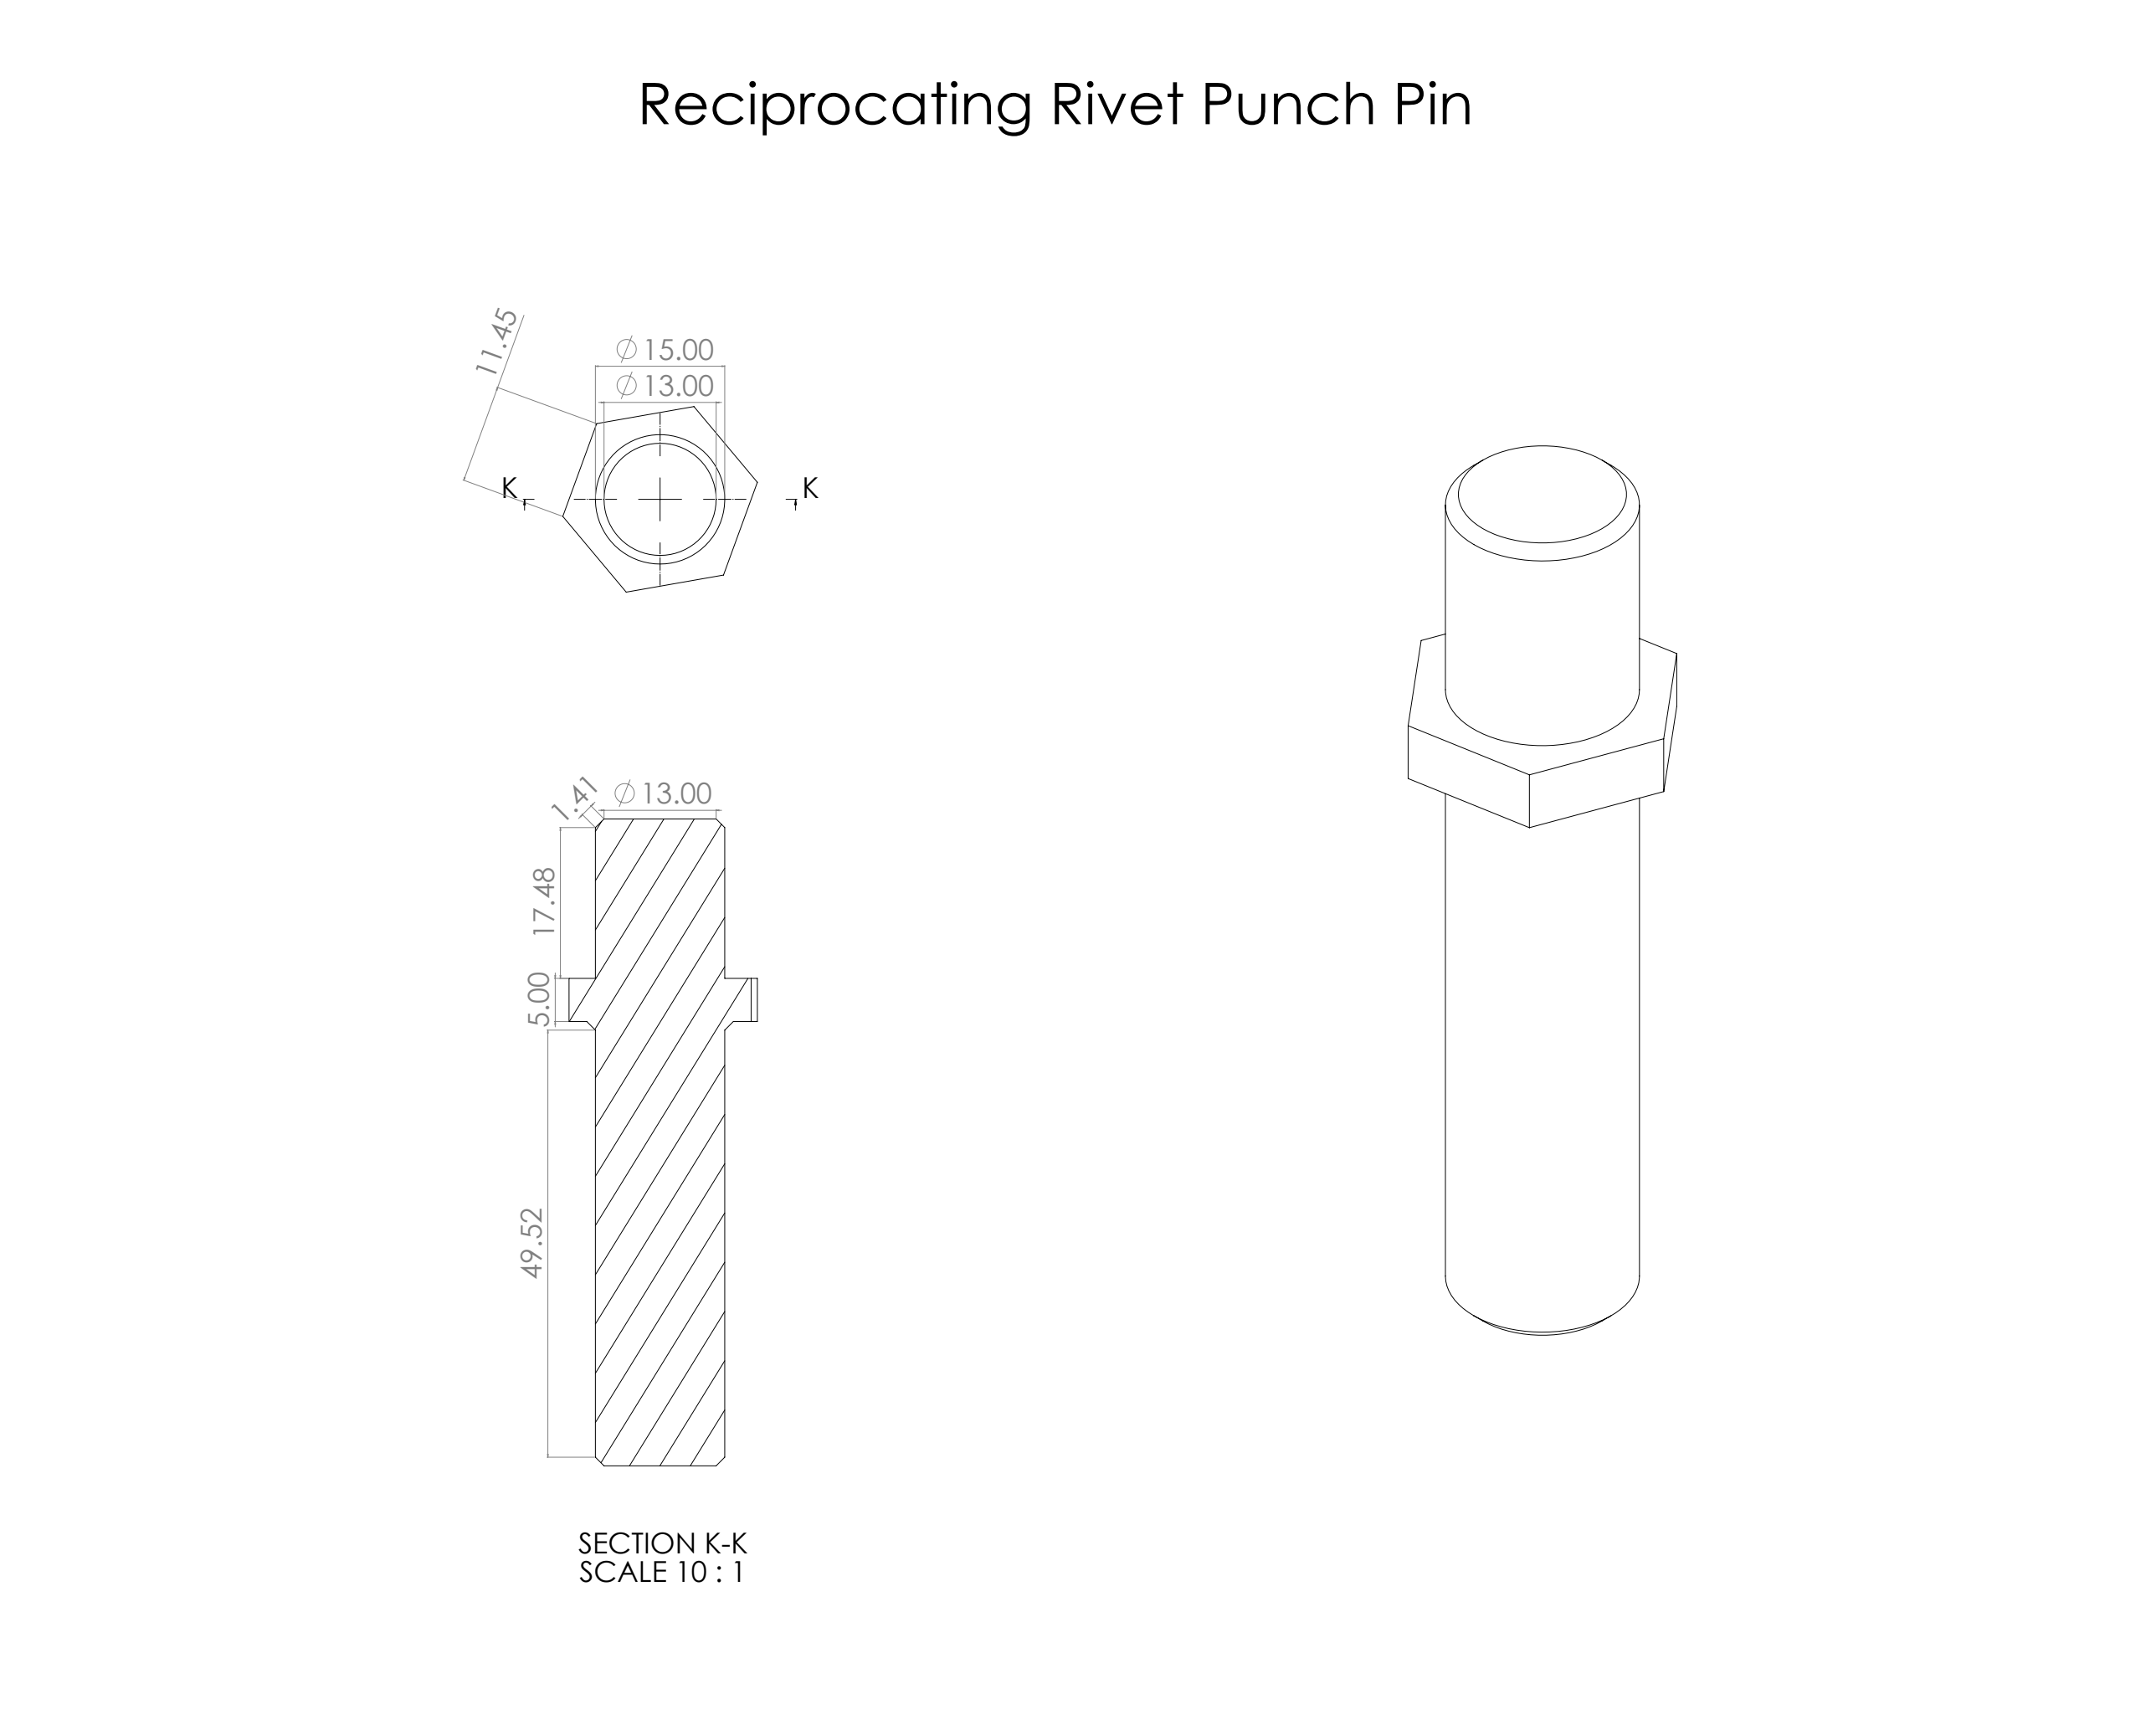
ISO-10303-21;
HEADER;
FILE_DESCRIPTION (('STEP AP214'),
    '1' );
FILE_NAME ('Reciprocating Rivet Punch Pin.step',
    '2026-10-25T20:52:49',
    ( '' ),
    ( '' ),
    'SwSTEP 2.0',
    'SolidWorks 2025',
    '' );
FILE_SCHEMA (( 'AUTOMOTIVE_DESIGN' ));
ENDSEC;

DATA;
#72=AXIS2_PLACEMENT_3D ( 'NONE', #82570, #38996, #88730 ) ;
#77=DIRECTION ( 'NONE',  ( -0.000000000000000000, 1.000000000000000000, -0.000000000000000000 ) ) ;
#121=DIRECTION ( 'NONE',  ( 0.000000000000000000, 0.7071067811865398012, 0.7071067811865552333 ) ) ;
#140=ADVANCED_BREP_SHAPE_REPRESENTATION ( '', ( #90135, #18940 ), #43137 ) ;
#206=PRODUCT_DEFINITION_CONTEXT ( 'detailed design', #57764, 'design' ) ;
#537=ORIENTED_EDGE ( 'NONE', *, *, #58978, .T. ) ;
#587=LINE ( 'NONE', #21899, #2031 ) ;
#976=EDGE_LOOP ( 'NONE', ( #39122, #15194, #45097, #86820 ) ) ;
#1223=FACE_OUTER_BOUND ( 'NONE', #24496, .T. ) ;
#1614=AXIS2_PLACEMENT_3D ( 'NONE', #18179, #47029, #23426 ) ;
#1655=EDGE_CURVE ( 'NONE', #7585, #19412, #71553, .T. ) ;
#1720=DIRECTION ( 'NONE',  ( 0.3428573139466625785, 0.000000000000000000, -0.9393874931428880526 ) ) ;
#1947=CARTESIAN_POINT ( 'NONE',  ( 208.4306832106270804, -199.2391364535880882, 0.000000000000000000 ) ) ;
#1975=DIRECTION ( 'NONE',  ( 0.000000000000000000, 0.000000000000000000, 1.000000000000000000 ) ) ;
#2031=VECTOR ( 'NONE', #28536, 1000.000000000000227 ) ;
#2392=MECHANICAL_DESIGN_GEOMETRIC_PRESENTATION_REPRESENTATION('',(#31117),#84023);
#2582=FACE_OUTER_BOUND ( 'NONE', #23796, .T. ) ;
#2617=ORIENTED_EDGE ( 'NONE', *, *, #23208, .F. ) ;
#2665=LINE ( 'NONE', #53304, #8085 ) ;
#2714=APPLICATION_CONTEXT ( 'automotive_design' ) ;
#2827=EDGE_LOOP ( 'NONE', ( #72963, #56833, #41843, #30949, #88679 ) ) ;
#3067=VERTEX_POINT ( 'NONE', #8877 ) ;
#3288=AXIS2_PLACEMENT_3D ( 'NONE', #82985, #37672, #54112 ) ;
#3409=EDGE_LOOP ( 'NONE', ( #92381, #68975, #16468, #27296, #33854 ) ) ;
#3425=AXIS2_PLACEMENT_3D ( 'NONE', #85327, #79169, #22323 ) ;
#3571=AXIS2_PLACEMENT_3D ( 'NONE', #21542, #6412, #86869 ) ;
#3656=CIRCLE ( 'NONE', #39922, 8.500000000000007105 ) ;
#3725=LINE ( 'NONE', #38757, #89716 ) ;
#3928=ORIENTED_EDGE ( 'NONE', *, *, #77906, .F. ) ;
#4091=FACE_OUTER_BOUND ( 'NONE', #61074, .T. ) ;
#4102=EDGE_CURVE ( 'NONE', #88194, #58673, #62613, .T. ) ;
#4316=AXIS2_PLACEMENT_3D ( 'NONE', #76033, #91140, #68939 ) ;
#4491=ADVANCED_FACE ( 'NONE', ( #1223 ), #8772, .T. ) ;
#4657=CIRCLE ( 'NONE', #63638, 7.500000000000012434 ) ;
#4770=EDGE_CURVE ( 'NONE', #55951, #76475, #59935, .T. ) ;
#4790=AXIS2_PLACEMENT_3D ( 'NONE', #49606, #85120, #20272 ) ;
#5162=FACE_OUTER_BOUND ( 'NONE', #92401, .T. ) ;
#5316=CLOSED_SHELL ( 'NONE', ( #16904, #77878, #27736, #81055, #54993, #32744, #82438, #11721, #85857, #23548, #86851, #61439, #15694, #44495, #51695, #4491, #81785, #83365, #7003, #77991 ) ) ;
#5328=CARTESIAN_POINT ( 'NONE',  ( 201.0776230153480526, -142.7221692137691775, -8.778910157967986905 ) ) ;
#5640=VERTEX_POINT ( 'NONE', #5328 ) ;
#5737=FACE_OUTER_BOUND ( 'NONE', #69469, .T. ) ;
#5766=VERTEX_POINT ( 'NONE', #42203 ) ;
#6030=EDGE_CURVE ( 'NONE', #93585, #33595, #3656, .T. ) ;
#6260=VERTEX_POINT ( 'NONE', #88559 ) ;
#6299=CIRCLE ( 'NONE', #4790, 7.500000000000012434 ) ;
#6412=DIRECTION ( 'NONE',  ( 0.000000000000000000, -1.000000000000000000, 0.000000000000000000 ) ) ;
#6560=CIRCLE ( 'NONE', #14137, 6.499999999999977796 ) ;
#6590=CIRCLE ( 'NONE', #11085, 7.500000000000012434 ) ;
#6657=CARTESIAN_POINT ( 'NONE',  ( 208.4306832106270804, -125.2391364535880882, -7.500000000000012434 ) ) ;
#6698=FACE_OUTER_BOUND ( 'NONE', #91473, .T. ) ;
#6794=DIRECTION ( 'NONE',  ( 8.659560562354937789E-17, -0.7071067811865472397, 0.7071067811865479058 ) ) ;
#7001=DIRECTION ( 'NONE',  ( 0.3428573139466625785, 0.000000000000000000, -0.9393874931428881636 ) ) ;
#7003=ADVANCED_FACE ( 'NONE', ( #25107 ), #30972, .T. ) ;
#7032=CARTESIAN_POINT ( 'NONE',  ( 208.4306832106270804, -124.2391364535881024, 6.500000000000033751 ) ) ;
#7127=DIRECTION ( 'NONE',  ( 0.000000000000000000, -1.000000000000000000, 0.000000000000000000 ) ) ;
#7130=DIRECTION ( 'NONE',  ( 0.000000000000000000, 0.7071067811865453523, 0.7071067811865496822 ) ) ;
#7541=EDGE_CURVE ( 'NONE', #54596, #88194, #59177, .T. ) ;
#7585=VERTEX_POINT ( 'NONE', #72013 ) ;
#7677=DIRECTION ( 'NONE',  ( 0.000000000000000000, -1.000000000000000000, 0.000000000000000000 ) ) ;
#7824=AXIS2_PLACEMENT_3D ( 'NONE', #80114, #7677, #30388 ) ;
#7846=CARTESIAN_POINT ( 'NONE',  ( 208.4306832106270804, -124.2391364535881024, 0.000000000000000000 ) ) ;
#8060=AXIS2_PLACEMENT_3D ( 'NONE', #85266, #71074, #64474 ) ;
#8085=VECTOR ( 'NONE', #1720, 1000.000000000000227 ) ;
#8088=SHAPE_REPRESENTATION_RELATIONSHIP ( 'NONE' , 'NONE' ,  #54338, #140 ) ;
#8356=DIRECTION ( 'NONE',  ( -0.9393874931428880526, 0.000000000000000000, -0.3428573139466629116 ) ) ;
#8384=PRODUCT_DEFINITION_FORMATION_WITH_SPECIFIED_SOURCE ( 'ANY', '', #15547, .NOT_KNOWN. ) ;
#8414=ORIENTED_EDGE ( 'NONE', *, *, #71951, .F. ) ;
#8515=LINE ( 'NONE', #80958, #86658 ) ;
#8772=PLANE ( 'NONE',  #50500 ) ;
#8877=CARTESIAN_POINT ( 'NONE',  ( 212.3569123273291268, -142.7221692137691775, -10.75739200365177695 ) ) ;
#9033=CYLINDRICAL_SURFACE ( 'NONE', #53545, 7.500000000000007105 ) ;
#9259=CARTESIAN_POINT ( 'NONE',  ( 208.4306832106270804, -124.2391364535881024, 0.000000000000000000 ) ) ;
#9285=EDGE_CURVE ( 'NONE', #6260, #33595, #40858, .T. ) ;
#9394=CARTESIAN_POINT ( 'NONE',  ( 204.5044540939250055, -147.7221692137691775, 10.75739200365177695 ) ) ;
#9436=DIRECTION ( 'NONE',  ( -1.000000000000000000, 0.000000000000000000, 0.000000000000000000 ) ) ;
#9489=CARTESIAN_POINT ( 'NONE',  ( 208.4306832106270804, -125.2391364535880882, 7.500000000000012434 ) ) ;
#9499=DIRECTION ( 'NONE',  ( -1.000000000000000000, 0.000000000000000000, 0.000000000000000000 ) ) ;
#9642=CIRCLE ( 'NONE', #62592, 6.500000000000033751 ) ;
#9668=CARTESIAN_POINT ( 'NONE',  ( 208.4306832106270804, -125.2391364535880882, 0.000000000000000000 ) ) ;
#9948=ORIENTED_EDGE ( 'NONE', *, *, #41512, .F. ) ;
#10028=DIRECTION ( 'NONE',  ( 0.1727706028203384314, 0.000000000000000000, 0.9849620900324524975 ) ) ;
#10210=DIRECTION ( 'NONE',  ( 1.124465274301078034E-16, 1.000000000000000000, 0.000000000000000000 ) ) ;
#10398=ORIENTED_EDGE ( 'NONE', *, *, #37113, .T. ) ;
#10664=EDGE_CURVE ( 'NONE', #76475, #64288, #20217, .T. ) ;
#10780=EDGE_CURVE ( 'NONE', #45114, #88143, #68943, .T. ) ;
#11003=ORIENTED_EDGE ( 'NONE', *, *, #10664, .F. ) ;
#11083=CYLINDRICAL_SURFACE ( 'NONE', #25795, 7.500000000000007105 ) ;
#11085=AXIS2_PLACEMENT_3D ( 'NONE', #46770, #69049, #68580 ) ;
#11101=VERTEX_POINT ( 'NONE', #43324 ) ;
#11263=EDGE_LOOP ( 'NONE', ( #75878, #62352 ) ) ;
#11601=UNCERTAINTY_MEASURE_WITH_UNIT (LENGTH_MEASURE( 1.000000000000000082E-05 ), #72501, 'distance_accuracy_value', 'NONE');
#11721=ADVANCED_FACE ( 'NONE', ( #12583, #14467 ), #20624, .T. ) ;
#11722=VERTEX_POINT ( 'NONE', #77439 ) ;
#12355=VERTEX_POINT ( 'NONE', #38848 ) ;
#12583=FACE_BOUND ( 'NONE', #70208, .T. ) ;
#12655=AXIS2_PLACEMENT_3D ( 'NONE', #19670, #75110, #76037 ) ;
#12972=EDGE_CURVE ( 'NONE', #34180, #5640, #63025, .T. ) ;
#13047=CARTESIAN_POINT ( 'NONE',  ( 215.9306832106270804, -199.2391364535880882, 9.184850993605165694E-16 ) ) ;
#13168=DIRECTION ( 'NONE',  ( -0.000000000000000000, 1.000000000000000000, -0.000000000000000000 ) ) ;
#13276=CARTESIAN_POINT ( 'NONE',  ( 208.4306832106270804, -147.7221692137691775, -8.500000000000007105 ) ) ;
#13304=LINE ( 'NONE', #27023, #54729 ) ;
#13606=CARTESIAN_POINT ( 'NONE',  ( 219.7099725226080977, -147.7221692137691775, -1.978481845683818907 ) ) ;
#13817=ORIENTED_EDGE ( 'NONE', *, *, #63823, .T. ) ;
#14137=AXIS2_PLACEMENT_3D ( 'NONE', #65588, #30978, #58466 ) ;
#14171=ORIENTED_EDGE ( 'NONE', *, *, #20803, .F. ) ;
#14349=DIRECTION ( 'NONE',  ( 0.000000000000000000, -1.000000000000000000, 0.000000000000000000 ) ) ;
#14467=FACE_OUTER_BOUND ( 'NONE', #66572, .T. ) ;
#14750=( NAMED_UNIT ( * ) SI_UNIT ( $, .STERADIAN. ) SOLID_ANGLE_UNIT ( ) );
#14841=CARTESIAN_POINT ( 'NONE',  ( 208.4306832106270804, -199.2391364535880882, -6.499999999999977796 ) ) ;
#14968=DIRECTION ( 'NONE',  ( -1.000000000000000000, 1.124465274301078034E-16, 0.000000000000000000 ) ) ;
#14996=ORIENTED_EDGE ( 'NONE', *, *, #71951, .T. ) ;
#15194=ORIENTED_EDGE ( 'NONE', *, *, #83604, .F. ) ;
#15469=CARTESIAN_POINT ( 'NONE',  ( 215.9306832106270804, -142.7221692137691775, 9.184850993605173582E-16 ) ) ;
#15547=PRODUCT ( 'Reciprocating Rivet Punch Pin', 'Reciprocating Rivet Punch Pin', '', ( #47307 ) ) ;
#15642=DIRECTION ( 'NONE',  ( -0.1727706028203382094, 0.000000000000000000, -0.9849620900324524975 ) ) ;
#15689=CARTESIAN_POINT ( 'NONE',  ( 200.9306832106270804, -198.2391364535880598, 0.000000000000000000 ) ) ;
#15694=ADVANCED_FACE ( 'NONE', ( #71880 ), #86979, .F. ) ;
#15702=VECTOR ( 'NONE', #13168, 1000.000000000000000 ) ;
#15862=EDGE_CURVE ( 'NONE', #33370, #72504, #6299, .T. ) ;
#16115=FACE_OUTER_BOUND ( 'NONE', #976, .T. ) ;
#16127=ORIENTED_EDGE ( 'NONE', *, *, #65170, .F. ) ;
#16202=CARTESIAN_POINT ( 'NONE',  ( 201.0776230153480526, -142.7221692137691775, -8.778910157967986905 ) ) ;
#16468=ORIENTED_EDGE ( 'NONE', *, *, #58978, .F. ) ;
#16556=DIRECTION ( 'NONE',  ( -0.9849620900324524975, 0.000000000000000000, 0.1727706028203382094 ) ) ;
#16904=ADVANCED_FACE ( 'NONE', ( #25374 ), #51681, .T. ) ;
#17060=ORIENTED_EDGE ( 'NONE', *, *, #41512, .T. ) ;
#17146=PLANE ( 'NONE',  #66255 ) ;
#17317=VECTOR ( 'NONE', #86922, 1000.000000000000227 ) ;
#17425=ORIENTED_EDGE ( 'NONE', *, *, #25604, .F. ) ;
#17781=CARTESIAN_POINT ( 'NONE',  ( 219.7099725226080977, -142.7221692137691775, -1.978481845683818907 ) ) ;
#17814=DIRECTION ( 'NONE',  ( 0.000000000000000000, 0.000000000000000000, -1.000000000000000000 ) ) ;
#17858=ORIENTED_EDGE ( 'NONE', *, *, #31125, .F. ) ;
#18014=DIRECTION ( 'NONE',  ( -0.6421047760857900855, 0.000000000000000000, -0.7666168903225504261 ) ) ;
#18179=CARTESIAN_POINT ( 'NONE',  ( 208.4306832106270804, -124.2391364535881024, 0.000000000000000000 ) ) ;
#18207=EDGE_CURVE ( 'NONE', #5766, #41385, #13304, .T. ) ;
#18488=DIRECTION ( 'NONE',  ( -0.000000000000000000, 1.000000000000000000, -0.000000000000000000 ) ) ;
#18617=CARTESIAN_POINT ( 'NONE',  ( 201.0776230153480526, -147.7221692137691775, -8.778910157967986905 ) ) ;
#18940=AXIS2_PLACEMENT_3D ( 'NONE', #90959, #40773, #33703 ) ;
#18953=ORIENTED_EDGE ( 'NONE', *, *, #91976, .T. ) ;
#19412=VERTEX_POINT ( 'NONE', #48154 ) ;
#19670=CARTESIAN_POINT ( 'NONE',  ( 208.4306832106270804, -198.2391364535880598, 0.000000000000000000 ) ) ;
#19762=ORIENTED_EDGE ( 'NONE', *, *, #42341, .T. ) ;
#20204=CARTESIAN_POINT ( 'NONE',  ( 208.4306832106270804, -198.2391364535880598, 0.000000000000000000 ) ) ;
#20217=CIRCLE ( 'NONE', #12655, 7.500000000000012434 ) ;
#20224=ORIENTED_EDGE ( 'NONE', *, *, #62141, .F. ) ;
#20272=DIRECTION ( 'NONE',  ( 0.000000000000000000, 0.000000000000000000, -1.000000000000000000 ) ) ;
#20412=VERTEX_POINT ( 'NONE', #23006 ) ;
#20624=PLANE ( 'NONE',  #3571 ) ;
#20706=ORIENTED_EDGE ( 'NONE', *, *, #63388, .F. ) ;
#20803=EDGE_CURVE ( 'NONE', #11722, #85835, #45229, .T. ) ;
#21161=DIRECTION ( 'NONE',  ( -0.3428573139466628561, 0.000000000000000000, 0.9393874931428880526 ) ) ;
#21282=ORIENTED_EDGE ( 'NONE', *, *, #58839, .F. ) ;
#21542=CARTESIAN_POINT ( 'NONE',  ( 0.000000000000000000, -147.7221692137691775, 0.000000000000000000 ) ) ;
#21704=VECTOR ( 'NONE', #54708, 1000.000000000000114 ) ;
#21849=( NAMED_UNIT ( * ) PLANE_ANGLE_UNIT ( ) SI_UNIT ( $, .RADIAN. ) );
#21899=CARTESIAN_POINT ( 'NONE',  ( 197.1513938986460062, -142.7221692137691775, 1.978481845683761620 ) ) ;
#22323=DIRECTION ( 'NONE',  ( 0.000000000000000000, 0.000000000000000000, -1.000000000000000000 ) ) ;
#22485=ORIENTED_EDGE ( 'NONE', *, *, #4102, .T. ) ;
#22559=DIRECTION ( 'NONE',  ( -0.3428573139466628561, 0.000000000000000000, 0.9393874931428879416 ) ) ;
#22606=LINE ( 'NONE', #73293, #53482 ) ;
#22911=EDGE_CURVE ( 'NONE', #58673, #7585, #52708, .T. ) ;
#23006=CARTESIAN_POINT ( 'NONE',  ( 215.9306832106270804, -125.2391364535880882, 9.184850993605173582E-16 ) ) ;
#23208=EDGE_CURVE ( 'NONE', #6260, #7585, #59410, .T. ) ;
#23426=DIRECTION ( 'NONE',  ( 0.000000000000000000, 0.000000000000000000, -1.000000000000000000 ) ) ;
#23548=ADVANCED_FACE ( 'NONE', ( #87872 ), #30599, .F. ) ;
#23558=EDGE_CURVE ( 'NONE', #3067, #11722, #66143, .T. ) ;
#23666=CARTESIAN_POINT ( 'NONE',  ( 208.4306832106270804, -199.2391364535880882, 0.000000000000000000 ) ) ;
#23796=EDGE_LOOP ( 'NONE', ( #2617, #58758, #77226, #53153, #79683 ) ) ;
#23934=EDGE_LOOP ( 'NONE', ( #17060, #22485, #26611, #77860, #537, #76910 ) ) ;
#24496=EDGE_LOOP ( 'NONE', ( #46361, #93472 ) ) ;
#24799=VECTOR ( 'NONE', #18488, 1000.000000000000000 ) ;
#24999=EDGE_CURVE ( 'NONE', #55951, #54596, #6560, .T. ) ;
#25002=CARTESIAN_POINT ( 'NONE',  ( 212.3569123273291268, -147.7221692137691775, -10.75739200365177695 ) ) ;
#25076=CARTESIAN_POINT ( 'NONE',  ( 215.7837434059060229, -147.7221692137691775, 8.778910157967997563 ) ) ;
#25083=CARTESIAN_POINT ( 'NONE',  ( 208.4306832106270804, -198.2391364535880598, 7.500000000000012434 ) ) ;
#25107=FACE_OUTER_BOUND ( 'NONE', #3409, .T. ) ;
#25374=FACE_OUTER_BOUND ( 'NONE', #46111, .T. ) ;
#25441=EDGE_LOOP ( 'NONE', ( #83264, #71223, #50033, #74140, #54424 ) ) ;
#25604=EDGE_CURVE ( 'NONE', #34180, #77042, #60786, .T. ) ;
#25730=CIRCLE ( 'NONE', #78678, 7.500000000000012434 ) ;
#25752=DIRECTION ( 'NONE',  ( -1.000000000000000000, 0.000000000000000000, 0.000000000000000000 ) ) ;
#25795=AXIS2_PLACEMENT_3D ( 'NONE', #61759, #90592, #25752 ) ;
#25846=DIRECTION ( 'NONE',  ( -0.6421047760857900855, 0.000000000000000000, -0.7666168903225505371 ) ) ;
#26204=VECTOR ( 'NONE', #91014, 1000.000000000000114 ) ;
#26611=ORIENTED_EDGE ( 'NONE', *, *, #22911, .T. ) ;
#26632=DIRECTION ( 'NONE',  ( 0.6421047760857910847, 0.000000000000000000, 0.7666168903225496489 ) ) ;
#26752=EDGE_CURVE ( 'NONE', #11101, #37419, #3725, .T. ) ;
#27023=CARTESIAN_POINT ( 'NONE',  ( 215.7837434059060229, -147.7221692137691775, 8.778910157967997563 ) ) ;
#27035=DIRECTION ( 'NONE',  ( 0.6421047760857910847, 0.000000000000000000, 0.7666168903225496489 ) ) ;
#27296=ORIENTED_EDGE ( 'NONE', *, *, #49214, .T. ) ;
#27646=VECTOR ( 'NONE', #73698, 1000.000000000000000 ) ;
#27736=ADVANCED_FACE ( 'NONE', ( #69867 ), #56315, .T. ) ;
#27854=DIRECTION ( 'NONE',  ( 0.9393874931428881636, 0.000000000000000000, 0.3428573139466625785 ) ) ;
#27980=DIRECTION ( 'NONE',  ( 0.000000000000000000, 0.000000000000000000, 1.000000000000000000 ) ) ;
#28464=PLANE ( 'NONE',  #35453 ) ;
#28536=DIRECTION ( 'NONE',  ( 0.3428573139466625785, 0.000000000000000000, -0.9393874931428880526 ) ) ;
#29004=CARTESIAN_POINT ( 'NONE',  ( 208.4306832106270804, -147.7221692137691775, 8.500000000000007105 ) ) ;
#30297=EDGE_CURVE ( 'NONE', #12355, #5766, #71369, .T. ) ;
#30388=DIRECTION ( 'NONE',  ( 0.000000000000000000, 0.000000000000000000, -1.000000000000000000 ) ) ;
#30404=LINE ( 'NONE', #16202, #63432 ) ;
#30467=ORIENTED_EDGE ( 'NONE', *, *, #4102, .F. ) ;
#30576=ORIENTED_EDGE ( 'NONE', *, *, #79173, .T. ) ;
#30590=DIRECTION ( 'NONE',  ( -1.000000000000000000, 0.000000000000000000, 0.000000000000000000 ) ) ;
#30599=PLANE ( 'NONE',  #41176 ) ;
#30783=AXIS2_PLACEMENT_3D ( 'NONE', #32164, #40168, #62940 ) ;
#30949=ORIENTED_EDGE ( 'NONE', *, *, #58839, .T. ) ;
#30972=CONICAL_SURFACE ( 'NONE', #65807, 8.500000000000007105, 0.7853981633974591592 ) ;
#30978=DIRECTION ( 'NONE',  ( -1.124465274301078034E-16, -1.000000000000000000, -0.000000000000000000 ) ) ;
#31117=STYLED_ITEM('',(#93752),#90135);
#31125=EDGE_CURVE ( 'NONE', #11101, #83213, #32020, .T. ) ;
#31483=CARTESIAN_POINT ( 'NONE',  ( 208.4306832106270804, -199.2391364535880882, 6.499999999999977796 ) ) ;
#31563=CIRCLE ( 'NONE', #4316, 7.500000000000012434 ) ;
#31615=ORIENTED_EDGE ( 'NONE', *, *, #12972, .T. ) ;
#31631=CARTESIAN_POINT ( 'NONE',  ( 201.0776230153480526, -147.7221692137691775, -8.778910157967986905 ) ) ;
#32020=CIRCLE ( 'NONE', #3288, 6.500000000000033751 ) ;
#32058=ORIENTED_EDGE ( 'NONE', *, *, #50406, .F. ) ;
#32164=CARTESIAN_POINT ( 'NONE',  ( 208.4306832106270804, -199.2391364535880882, 0.000000000000000000 ) ) ;
#32602=CARTESIAN_POINT ( 'NONE',  ( 197.1513938986460062, -147.7221692137691775, 1.978481845683761620 ) ) ;
#32744=ADVANCED_FACE ( 'NONE', ( #73916 ), #9033, .T. ) ;
#32799=LINE ( 'NONE', #90984, #60892 ) ;
#32962=PLANE ( 'NONE',  #72925 ) ;
#32977=ORIENTED_EDGE ( 'NONE', *, *, #20803, .T. ) ;
#33171=CARTESIAN_POINT ( 'NONE',  ( 208.4306832106270804, -147.7221692137691775, 0.000000000000000000 ) ) ;
#33370=VERTEX_POINT ( 'NONE', #48284 ) ;
#33595=VERTEX_POINT ( 'NONE', #13276 ) ;
#33703=DIRECTION ( 'NONE',  ( 1.000000000000000000, 0.000000000000000000, 0.000000000000000000 ) ) ;
#33854=ORIENTED_EDGE ( 'NONE', *, *, #37113, .F. ) ;
#34037=PLANE ( 'NONE',  #30783 ) ;
#34180=VERTEX_POINT ( 'NONE', #31631 ) ;
#34838=CARTESIAN_POINT ( 'NONE',  ( 208.4306832106270804, -199.2391364535880882, 0.000000000000000000 ) ) ;
#35128=EDGE_LOOP ( 'NONE', ( #52939, #84957, #51732, #30467, #80366 ) ) ;
#35370=AXIS2_PLACEMENT_3D ( 'NONE', #20204, #49083, #77981 ) ;
#35382=AXIS2_PLACEMENT_3D ( 'NONE', #58618, #79915, #67115 ) ;
#35453=AXIS2_PLACEMENT_3D ( 'NONE', #50704, #79592, #36028 ) ;
#35595=ORIENTED_EDGE ( 'NONE', *, *, #4770, .F. ) ;
#35872=EDGE_CURVE ( 'NONE', #88143, #5640, #587, .T. ) ;
#36028=DIRECTION ( 'NONE',  ( 0.000000000000000000, -0.000000000000000000, -1.000000000000000000 ) ) ;
#36222=CIRCLE ( 'NONE', #70980, 7.500000000000012434 ) ;
#36420=ORIENTED_EDGE ( 'NONE', *, *, #24999, .T. ) ;
#36556=CIRCLE ( 'NONE', #84942, 7.500000000000012434 ) ;
#36765=DIRECTION ( 'NONE',  ( 1.124465274301078034E-16, 1.000000000000000000, 0.000000000000000000 ) ) ;
#37113=EDGE_CURVE ( 'NONE', #33595, #93585, #74616, .T. ) ;
#37419=VERTEX_POINT ( 'NONE', #6657 ) ;
#37672=DIRECTION ( 'NONE',  ( 1.124465274301078034E-16, 1.000000000000000000, 0.000000000000000000 ) ) ;
#37692=LINE ( 'NONE', #75100, #45859 ) ;
#38198=ORIENTED_EDGE ( 'NONE', *, *, #25604, .T. ) ;
#38757=CARTESIAN_POINT ( 'NONE',  ( 208.4306832106270804, -124.2391364535881024, -6.500000000000024869 ) ) ;
#38848=CARTESIAN_POINT ( 'NONE',  ( 219.7099725226080977, -147.7221692137691775, -1.978481845683818907 ) ) ;
#38869=CARTESIAN_POINT ( 'NONE',  ( 208.4306832106270804, -125.2391364535880882, 0.000000000000000000 ) ) ;
#38898=DIRECTION ( 'NONE',  ( 0.9849620900324523864, 0.000000000000000000, -0.1727706028203384037 ) ) ;
#38996=DIRECTION ( 'NONE',  ( -0.000000000000000000, 1.000000000000000000, -0.000000000000000000 ) ) ;
#39059=DIRECTION ( 'NONE',  ( -0.3428573139466628561, 0.000000000000000000, 0.9393874931428880526 ) ) ;
#39122=ORIENTED_EDGE ( 'NONE', *, *, #81466, .T. ) ;
#39171=DIRECTION ( 'NONE',  ( -0.000000000000000000, 1.000000000000000000, -0.000000000000000000 ) ) ;
#39359=CONICAL_SURFACE ( 'NONE', #72, 8.500000000000007105, 0.7853981633974591592 ) ;
#39455=FACE_OUTER_BOUND ( 'NONE', #75250, .T. ) ;
#39550=CARTESIAN_POINT ( 'NONE',  ( 208.4306832106270804, -124.2391364535881024, 0.000000000000000000 ) ) ;
#39922=AXIS2_PLACEMENT_3D ( 'NONE', #64974, #77, #88080 ) ;
#40000=AXIS2_PLACEMENT_3D ( 'NONE', #25076, #15642, #59204 ) ;
#40032=DIRECTION ( 'NONE',  ( 0.000000000000000000, -1.000000000000000000, 0.000000000000000000 ) ) ;
#40168=DIRECTION ( 'NONE',  ( 1.124465274301078034E-16, 1.000000000000000000, 0.000000000000000000 ) ) ;
#40188=DIRECTION ( 'NONE',  ( 0.000000000000000000, 0.000000000000000000, -1.000000000000000000 ) ) ;
#40526=UNCERTAINTY_MEASURE_WITH_UNIT (LENGTH_MEASURE( 1.000000000000000082E-05 ), #42925, 'distance_accuracy_value', 'NONE');
#40649=CARTESIAN_POINT ( 'NONE',  ( 197.1513938986460062, -142.7221692137691775, 1.978481845683761620 ) ) ;
#40773=DIRECTION ( 'NONE',  ( 0.000000000000000000, 0.000000000000000000, 1.000000000000000000 ) ) ;
#40858=LINE ( 'NONE', #75475, #59487 ) ;
#41175=DIRECTION ( 'NONE',  ( 0.000000000000000000, 0.000000000000000000, -1.000000000000000000 ) ) ;
#41176=AXIS2_PLACEMENT_3D ( 'NONE', #73245, #8356, #22559 ) ;
#41289=DIRECTION ( 'NONE',  ( 0.000000000000000000, 0.000000000000000000, -1.000000000000000000 ) ) ;
#41385=VERTEX_POINT ( 'NONE', #9394 ) ;
#41512=EDGE_CURVE ( 'NONE', #64288, #88194, #6590, .T. ) ;
#41552=VECTOR ( 'NONE', #7130, 1000.000000000000227 ) ;
#41624=EDGE_CURVE ( 'NONE', #72504, #33370, #86650, .T. ) ;
#41843=ORIENTED_EDGE ( 'NONE', *, *, #77906, .T. ) ;
#42203=CARTESIAN_POINT ( 'NONE',  ( 215.7837434059060229, -147.7221692137691775, 8.778910157967997563 ) ) ;
#42341=EDGE_CURVE ( 'NONE', #12355, #11722, #78028, .T. ) ;
#42925=( LENGTH_UNIT ( ) NAMED_UNIT ( * ) SI_UNIT ( .MILLI., .METRE. ) );
#43137=( GEOMETRIC_REPRESENTATION_CONTEXT ( 3 ) GLOBAL_UNCERTAINTY_ASSIGNED_CONTEXT ( ( #11601 ) ) GLOBAL_UNIT_ASSIGNED_CONTEXT ( ( #72501, #21849, #14750 ) ) REPRESENTATION_CONTEXT ( 'NONE', 'WORKASPACE' ) );
#43211=LINE ( 'NONE', #29004, #58810 ) ;
#43324=CARTESIAN_POINT ( 'NONE',  ( 208.4306832106270804, -124.2391364535881024, -6.500000000000033751 ) ) ;
#43487=DIRECTION ( 'NONE',  ( -0.000000000000000000, 1.000000000000000000, -0.000000000000000000 ) ) ;
#43625=EDGE_LOOP ( 'NONE', ( #50959, #20224, #17425, #31615 ) ) ;
#44040=FACE_BOUND ( 'NONE', #11263, .T. ) ;
#44114=AXIS2_PLACEMENT_3D ( 'NONE', #92685, #27854, #7001 ) ;
#44495=ADVANCED_FACE ( 'NONE', ( #73969 ), #17146, .F. ) ;
#44749=VECTOR ( 'NONE', #43487, 1000.000000000000000 ) ;
#44966=PLANE ( 'NONE',  #40000 ) ;
#45097=ORIENTED_EDGE ( 'NONE', *, *, #18207, .F. ) ;
#45114=VERTEX_POINT ( 'NONE', #68746 ) ;
#45229=LINE ( 'NONE', #17781, #77447 ) ;
#45323=EDGE_CURVE ( 'NONE', #33370, #62133, #87134, .T. ) ;
#45592=DIRECTION ( 'NONE',  ( 1.124465274301078034E-16, 1.000000000000000000, 0.000000000000000000 ) ) ;
#45787=VECTOR ( 'NONE', #45592, 1000.000000000000000 ) ;
#45859=VECTOR ( 'NONE', #10210, 1000.000000000000000 ) ;
#45922=SHAPE_DEFINITION_REPRESENTATION ( #58649, #54338 ) ;
#46013=CARTESIAN_POINT ( 'NONE',  ( 201.0776230153480526, -147.7221692137691775, -8.778910157967986905 ) ) ;
#46111=EDGE_LOOP ( 'NONE', ( #90811, #30576, #3928, #90125, #72298 ) ) ;
#46238=ORIENTED_EDGE ( 'NONE', *, *, #10780, .F. ) ;
#46295=ORIENTED_EDGE ( 'NONE', *, *, #49739, .F. ) ;
#46361=ORIENTED_EDGE ( 'NONE', *, *, #31125, .T. ) ;
#46453=ORIENTED_EDGE ( 'NONE', *, *, #7541, .T. ) ;
#46714=EDGE_CURVE ( 'NONE', #58673, #76475, #31563, .T. ) ;
#46770=CARTESIAN_POINT ( 'NONE',  ( 208.4306832106270804, -198.2391364535880598, 0.000000000000000000 ) ) ;
#47029=DIRECTION ( 'NONE',  ( 0.000000000000000000, -1.000000000000000000, 0.000000000000000000 ) ) ;
#47307=PRODUCT_CONTEXT ( 'NONE', #2714, 'mechanical' ) ;
#47339=VECTOR ( 'NONE', #18014, 1000.000000000000114 ) ;
#47366=AXIS2_PLACEMENT_3D ( 'NONE', #23666, #52075, #9436 ) ;
#47991=LINE ( 'NONE', #71208, #83307 ) ;
#48116=ORIENTED_EDGE ( 'NONE', *, *, #18207, .T. ) ;
#48154=CARTESIAN_POINT ( 'NONE',  ( 208.4306832106270804, -148.7221692137691491, 7.500000000000012434 ) ) ;
#48159=EDGE_LOOP ( 'NONE', ( #60231, #58105, #8414, #18953 ) ) ;
#48284=CARTESIAN_POINT ( 'NONE',  ( 200.9306832106270804, -142.7221692137691775, 0.000000000000000000 ) ) ;
#48300=AXIS2_PLACEMENT_3D ( 'NONE', #34838, #92114, #56155 ) ;
#48462=DIRECTION ( 'NONE',  ( -0.000000000000000000, 1.000000000000000000, -0.000000000000000000 ) ) ;
#48537=DIRECTION ( 'NONE',  ( -0.000000000000000000, 1.000000000000000000, -0.000000000000000000 ) ) ;
#49083=DIRECTION ( 'NONE',  ( -0.000000000000000000, 1.000000000000000000, -0.000000000000000000 ) ) ;
#49214=EDGE_CURVE ( 'NONE', #19412, #93585, #43211, .T. ) ;
#49283=FACE_OUTER_BOUND ( 'NONE', #2827, .T. ) ;
#49606=CARTESIAN_POINT ( 'NONE',  ( 208.4306832106270804, -142.7221692137691775, 0.000000000000000000 ) ) ;
#49675=EDGE_LOOP ( 'NONE', ( #35595, #32058, #46453, #9948, #11003 ) ) ;
#49739=EDGE_CURVE ( 'NONE', #62133, #37419, #36222, .T. ) ;
#50033=ORIENTED_EDGE ( 'NONE', *, *, #45323, .T. ) ;
#50300=CARTESIAN_POINT ( 'NONE',  ( 215.9306832106270804, -198.2391364535880598, 9.184850993605173582E-16 ) ) ;
#50339=AXIS2_PLACEMENT_3D ( 'NONE', #62660, #90091, #41289 ) ;
#50406=EDGE_CURVE ( 'NONE', #54596, #55951, #92104, .T. ) ;
#50500=AXIS2_PLACEMENT_3D ( 'NONE', #7846, #65189, #14968 ) ;
#50704=CARTESIAN_POINT ( 'NONE',  ( 0.000000000000000000, -142.7221692137691775, 0.000000000000000000 ) ) ;
#50727=ORIENTED_EDGE ( 'NONE', *, *, #91976, .F. ) ;
#50919=EDGE_CURVE ( 'NONE', #5640, #3067, #30404, .T. ) ;
#50959=ORIENTED_EDGE ( 'NONE', *, *, #50919, .T. ) ;
#51133=CARTESIAN_POINT ( 'NONE',  ( 208.4306832106270804, -198.2391364535880598, 7.500000000000012434 ) ) ;
#51242=DIRECTION ( 'NONE',  ( 0.9849620900324523864, 0.000000000000000000, -0.1727706028203384037 ) ) ;
#51681=CONICAL_SURFACE ( 'NONE', #75964, 6.500000000000024869, 0.7853981633974488341 ) ;
#51695=ADVANCED_FACE ( 'NONE', ( #5737 ), #64931, .F. ) ;
#51732=ORIENTED_EDGE ( 'NONE', *, *, #46714, .F. ) ;
#51989=ORIENTED_EDGE ( 'NONE', *, *, #62141, .T. ) ;
#52075=DIRECTION ( 'NONE',  ( 1.124465274301078034E-16, 1.000000000000000000, 0.000000000000000000 ) ) ;
#52423=DIRECTION ( 'NONE',  ( -0.000000000000000000, 1.000000000000000000, -0.000000000000000000 ) ) ;
#52708=LINE ( 'NONE', #66483, #45787 ) ;
#52939=ORIENTED_EDGE ( 'NONE', *, *, #24999, .F. ) ;
#53153=ORIENTED_EDGE ( 'NONE', *, *, #49214, .F. ) ;
#53304=CARTESIAN_POINT ( 'NONE',  ( 197.1513938986460062, -147.7221692137691775, 1.978481845683761620 ) ) ;
#53482=VECTOR ( 'NONE', #52423, 1000.000000000000000 ) ;
#53545=AXIS2_PLACEMENT_3D ( 'NONE', #1947, #89032, #9499 ) ;
#53981=CARTESIAN_POINT ( 'NONE',  ( 208.4306832106270804, -147.7221692137691775, 0.000000000000000000 ) ) ;
#53993=CARTESIAN_POINT ( 'NONE',  ( 204.5044540939250055, -147.7221692137691775, 10.75739200365177695 ) ) ;
#54070=ORIENTED_EDGE ( 'NONE', *, *, #6030, .T. ) ;
#54112=DIRECTION ( 'NONE',  ( -1.000000000000000000, 0.000000000000000000, 0.000000000000000000 ) ) ;
#54249=CARTESIAN_POINT ( 'NONE',  ( 204.5044540939250055, -142.7221692137691775, 10.75739200365177695 ) ) ;
#54338=SHAPE_REPRESENTATION ( 'Reciprocating Rivet Punch Pin', ( #18940 ), #43137 ) ;
#54424=ORIENTED_EDGE ( 'NONE', *, *, #76676, .T. ) ;
#54596=VERTEX_POINT ( 'NONE', #31483 ) ;
#54708=DIRECTION ( 'NONE',  ( -0.6421047760857900855, 0.000000000000000000, -0.7666168903225504261 ) ) ;
#54729=VECTOR ( 'NONE', #61615, 1000.000000000000000 ) ;
#54993=ADVANCED_FACE ( 'NONE', ( #75951 ), #11083, .T. ) ;
#55385=ORIENTED_EDGE ( 'NONE', *, *, #23208, .T. ) ;
#55554=EDGE_CURVE ( 'NONE', #5766, #85835, #47991, .T. ) ;
#55951=VERTEX_POINT ( 'NONE', #14841 ) ;
#56155=DIRECTION ( 'NONE',  ( -1.000000000000000000, 0.000000000000000000, 0.000000000000000000 ) ) ;
#56315=CONICAL_SURFACE ( 'NONE', #77525, 7.500000000000012434, 0.7853981633974513876 ) ;
#56593=VECTOR ( 'NONE', #91610, 1000.000000000000000 ) ;
#56729=CARTESIAN_POINT ( 'NONE',  ( 219.7099725226080977, -147.7221692137691775, -1.978481845683818907 ) ) ;
#56833=ORIENTED_EDGE ( 'NONE', *, *, #68323, .T. ) ;
#57764=APPLICATION_CONTEXT ( 'automotive_design' ) ;
#57889=VECTOR ( 'NONE', #6794, 1000.000000000000000 ) ;
#57959=AXIS2_PLACEMENT_3D ( 'NONE', #61941, #69979, #62417 ) ;
#58068=CARTESIAN_POINT ( 'NONE',  ( 208.4306832106270804, -198.2391364535880598, -7.500000000000012434 ) ) ;
#58105=ORIENTED_EDGE ( 'NONE', *, *, #12972, .F. ) ;
#58466=DIRECTION ( 'NONE',  ( -1.000000000000000000, 0.000000000000000000, 0.000000000000000000 ) ) ;
#58618=CARTESIAN_POINT ( 'NONE',  ( 208.4306832106270804, -198.2391364535880598, 0.000000000000000000 ) ) ;
#58649=PRODUCT_DEFINITION_SHAPE ( 'NONE', 'NONE',  #69577 ) ;
#58673=VERTEX_POINT ( 'NONE', #50300 ) ;
#58758=ORIENTED_EDGE ( 'NONE', *, *, #9285, .T. ) ;
#58810=VECTOR ( 'NONE', #121, 1000.000000000000114 ) ;
#58839=EDGE_CURVE ( 'NONE', #64509, #62133, #36556, .T. ) ;
#58978=EDGE_CURVE ( 'NONE', #19412, #90166, #87966, .T. ) ;
#59177=LINE ( 'NONE', #51133, #41552 ) ;
#59204=DIRECTION ( 'NONE',  ( -0.9849620900324524975, 0.000000000000000000, 0.1727706028203382094 ) ) ;
#59282=DIRECTION ( 'NONE',  ( 0.000000000000000000, -1.000000000000000000, 0.000000000000000000 ) ) ;
#59410=CIRCLE ( 'NONE', #50339, 7.500000000000012434 ) ;
#59487=VECTOR ( 'NONE', #67913, 1000.000000000000114 ) ;
#59554=FACE_OUTER_BOUND ( 'NONE', #49675, .T. ) ;
#59588=CONICAL_SURFACE ( 'NONE', #35382, 7.500000000000012434, 0.7853981633974513876 ) ;
#59935=LINE ( 'NONE', #58068, #17317 ) ;
#60230=VECTOR ( 'NONE', #86666, 1000.000000000000000 ) ;
#60231=ORIENTED_EDGE ( 'NONE', *, *, #35872, .T. ) ;
#60594=CYLINDRICAL_SURFACE ( 'NONE', #47366, 7.500000000000007105 ) ;
#60786=LINE ( 'NONE', #18617, #26204 ) ;
#60892=VECTOR ( 'NONE', #26632, 1000.000000000000000 ) ;
#61074=EDGE_LOOP ( 'NONE', ( #66199, #50727, #16127, #84816 ) ) ;
#61325=ORIENTED_EDGE ( 'NONE', *, *, #63388, .T. ) ;
#61439=ADVANCED_FACE ( 'NONE', ( #4091 ), #32962, .F. ) ;
#61615=DIRECTION ( 'NONE',  ( -0.9849620900324524975, 0.000000000000000000, 0.1727706028203382094 ) ) ;
#61668=ORIENTED_EDGE ( 'NONE', *, *, #26752, .T. ) ;
#61759=CARTESIAN_POINT ( 'NONE',  ( 208.4306832106270804, -199.2391364535880882, 0.000000000000000000 ) ) ;
#61855=CARTESIAN_POINT ( 'NONE',  ( 204.5044540939250055, -147.7221692137691775, 10.75739200365177695 ) ) ;
#61941=CARTESIAN_POINT ( 'NONE',  ( 208.4306832106270804, -142.7221692137691775, 0.000000000000000000 ) ) ;
#62061=DIRECTION ( 'NONE',  ( -0.000000000000000000, 1.000000000000000000, -0.000000000000000000 ) ) ;
#62133=VERTEX_POINT ( 'NONE', #68552 ) ;
#62141=EDGE_CURVE ( 'NONE', #77042, #3067, #75646, .T. ) ;
#62189=ORIENTED_EDGE ( 'NONE', *, *, #23558, .T. ) ;
#62352=ORIENTED_EDGE ( 'NONE', *, *, #41624, .T. ) ;
#62417=DIRECTION ( 'NONE',  ( 0.000000000000000000, 0.000000000000000000, -1.000000000000000000 ) ) ;
#62592=AXIS2_PLACEMENT_3D ( 'NONE', #9259, #36765, #30590 ) ;
#62613=CIRCLE ( 'NONE', #35370, 7.500000000000012434 ) ;
#62660=CARTESIAN_POINT ( 'NONE',  ( 208.4306832106270804, -148.7221692137691491, 0.000000000000000000 ) ) ;
#62940=DIRECTION ( 'NONE',  ( -1.000000000000000000, 1.124465274301078034E-16, 0.000000000000000000 ) ) ;
#63025=LINE ( 'NONE', #76269, #24799 ) ;
#63388=EDGE_CURVE ( 'NONE', #77042, #12355, #32799, .T. ) ;
#63432=VECTOR ( 'NONE', #51242, 1000.000000000000114 ) ;
#63638=AXIS2_PLACEMENT_3D ( 'NONE', #9668, #67908, #74069 ) ;
#63673=ORIENTED_EDGE ( 'NONE', *, *, #65170, .T. ) ;
#63823=EDGE_CURVE ( 'NONE', #90166, #6260, #65515, .T. ) ;
#64288=VERTEX_POINT ( 'NONE', #15689 ) ;
#64471=ORIENTED_EDGE ( 'NONE', *, *, #10664, .T. ) ;
#64474=DIRECTION ( 'NONE',  ( -1.000000000000000000, 0.000000000000000000, 0.000000000000000000 ) ) ;
#64509=VERTEX_POINT ( 'NONE', #9489 ) ;
#64744=CARTESIAN_POINT ( 'NONE',  ( 200.9306832106270804, -148.7221692137691491, 0.000000000000000000 ) ) ;
#64863=ORIENTED_EDGE ( 'NONE', *, *, #42341, .F. ) ;
#64931=PLANE ( 'NONE',  #68055 ) ;
#64974=CARTESIAN_POINT ( 'NONE',  ( 208.4306832106270804, -147.7221692137691775, 0.000000000000000000 ) ) ;
#65170=EDGE_CURVE ( 'NONE', #41385, #71100, #77178, .T. ) ;
#65189=DIRECTION ( 'NONE',  ( 1.124465274301078034E-16, 1.000000000000000000, 0.000000000000000000 ) ) ;
#65515=CIRCLE ( 'NONE', #3425, 7.500000000000012434 ) ;
#65588=CARTESIAN_POINT ( 'NONE',  ( 208.4306832106270804, -199.2391364535880882, 0.000000000000000000 ) ) ;
#65807=AXIS2_PLACEMENT_3D ( 'NONE', #53981, #83312, #82850 ) ;
#66135=ORIENTED_EDGE ( 'NONE', *, *, #35872, .F. ) ;
#66143=LINE ( 'NONE', #67986, #27646 ) ;
#66199=ORIENTED_EDGE ( 'NONE', *, *, #10780, .T. ) ;
#66255=AXIS2_PLACEMENT_3D ( 'NONE', #46013, #10028, #38898 ) ;
#66483=CARTESIAN_POINT ( 'NONE',  ( 215.9306832106270804, -199.2391364535880882, 9.184850993605165694E-16 ) ) ;
#66572=EDGE_LOOP ( 'NONE', ( #69188, #48116, #63673, #14996, #38198, #61325 ) ) ;
#66764=EDGE_LOOP ( 'NONE', ( #90459, #73802, #64471, #88072, #13817, #55385 ) ) ;
#67115=DIRECTION ( 'NONE',  ( 0.000000000000000000, 0.000000000000000000, 1.000000000000000000 ) ) ;
#67295=EDGE_CURVE ( 'NONE', #83213, #11101, #9642, .T. ) ;
#67661=DIRECTION ( 'NONE',  ( 0.000000000000000000, -0.7071067811865472397, -0.7071067811865479058 ) ) ;
#67908=DIRECTION ( 'NONE',  ( 0.000000000000000000, -1.000000000000000000, 0.000000000000000000 ) ) ;
#67913=DIRECTION ( 'NONE',  ( 8.659560562355027768E-17, 0.7071067811865398012, -0.7071067811865552333 ) ) ;
#67986=CARTESIAN_POINT ( 'NONE',  ( 212.3569123273291268, -142.7221692137691775, -10.75739200365177695 ) ) ;
#68055=AXIS2_PLACEMENT_3D ( 'NONE', #78640, #84776, #27035 ) ;
#68323=EDGE_CURVE ( 'NONE', #72504, #20412, #70342, .T. ) ;
#68552=CARTESIAN_POINT ( 'NONE',  ( 200.9306832106270804, -125.2391364535880882, 0.000000000000000000 ) ) ;
#68580=DIRECTION ( 'NONE',  ( 0.000000000000000000, 0.000000000000000000, 1.000000000000000000 ) ) ;
#68746=CARTESIAN_POINT ( 'NONE',  ( 204.5044540939250055, -142.7221692137691775, 10.75739200365177695 ) ) ;
#68939=DIRECTION ( 'NONE',  ( 0.000000000000000000, 0.000000000000000000, 1.000000000000000000 ) ) ;
#68943=LINE ( 'NONE', #54249, #21704 ) ;
#68975=ORIENTED_EDGE ( 'NONE', *, *, #63823, .F. ) ;
#69049=DIRECTION ( 'NONE',  ( -0.000000000000000000, 1.000000000000000000, -0.000000000000000000 ) ) ;
#69188=ORIENTED_EDGE ( 'NONE', *, *, #30297, .T. ) ;
#69469=EDGE_LOOP ( 'NONE', ( #62189, #64863, #20706, #51989 ) ) ;
#69577=PRODUCT_DEFINITION ( 'UNKNOWN', '', #8384, #206 ) ;
#69867=FACE_OUTER_BOUND ( 'NONE', #35128, .T. ) ;
#69979=DIRECTION ( 'NONE',  ( 0.000000000000000000, -1.000000000000000000, 0.000000000000000000 ) ) ;
#70017=VECTOR ( 'NONE', #39171, 1000.000000000000000 ) ;
#70208=EDGE_LOOP ( 'NONE', ( #54070, #10398 ) ) ;
#70342=LINE ( 'NONE', #13047, #56593 ) ;
#70980=AXIS2_PLACEMENT_3D ( 'NONE', #38869, #59282, #1975 ) ;
#71074=DIRECTION ( 'NONE',  ( 1.124465274301078034E-16, 1.000000000000000000, 0.000000000000000000 ) ) ;
#71100=VERTEX_POINT ( 'NONE', #32602 ) ;
#71208=CARTESIAN_POINT ( 'NONE',  ( 215.7837434059060229, -147.7221692137691775, 8.778910157967997563 ) ) ;
#71223=ORIENTED_EDGE ( 'NONE', *, *, #15862, .F. ) ;
#71369=LINE ( 'NONE', #13606, #87964 ) ;
#71487=AXIS2_PLACEMENT_3D ( 'NONE', #77139, #76670, #40188 ) ;
#71553=CIRCLE ( 'NONE', #71487, 7.500000000000012434 ) ;
#71880=FACE_OUTER_BOUND ( 'NONE', #48159, .T. ) ;
#71951=EDGE_CURVE ( 'NONE', #71100, #34180, #2665, .T. ) ;
#72010=CARTESIAN_POINT ( 'NONE',  ( 208.4306832106270804, -125.2391364535880882, 0.000000000000000000 ) ) ;
#72013=CARTESIAN_POINT ( 'NONE',  ( 215.9306832106270804, -148.7221692137691491, 9.184850993605173582E-16 ) ) ;
#72298=ORIENTED_EDGE ( 'NONE', *, *, #26752, .F. ) ;
#72465=EDGE_CURVE ( 'NONE', #64288, #90166, #37692, .T. ) ;
#72484=CARTESIAN_POINT ( 'NONE',  ( 215.7837434059060229, -142.7221692137691775, 8.778910157967997563 ) ) ;
#72501=( LENGTH_UNIT ( ) NAMED_UNIT ( * ) SI_UNIT ( .MILLI., .METRE. ) );
#72504=VERTEX_POINT ( 'NONE', #15469 ) ;
#72574=CARTESIAN_POINT ( 'NONE',  ( 208.4306832106270804, -124.2391364535881024, 6.500000000000024869 ) ) ;
#72925=AXIS2_PLACEMENT_3D ( 'NONE', #61855, #90686, #25846 ) ;
#72963=ORIENTED_EDGE ( 'NONE', *, *, #41624, .F. ) ;
#73245=CARTESIAN_POINT ( 'NONE',  ( 219.7099725226080977, -147.7221692137691775, -1.978481845683818907 ) ) ;
#73293=CARTESIAN_POINT ( 'NONE',  ( 204.5044540939250055, -147.7221692137691775, 10.75739200365177695 ) ) ;
#73541=ORIENTED_EDGE ( 'NONE', *, *, #55554, .F. ) ;
#73698=DIRECTION ( 'NONE',  ( 0.6421047760857910847, 0.000000000000000000, 0.7666168903225496489 ) ) ;
#73802=ORIENTED_EDGE ( 'NONE', *, *, #46714, .T. ) ;
#73916=FACE_OUTER_BOUND ( 'NONE', #66764, .T. ) ;
#73969=FACE_OUTER_BOUND ( 'NONE', #43625, .T. ) ;
#74069=DIRECTION ( 'NONE',  ( 0.000000000000000000, 0.000000000000000000, 1.000000000000000000 ) ) ;
#74140=ORIENTED_EDGE ( 'NONE', *, *, #49739, .T. ) ;
#74201=CONICAL_SURFACE ( 'NONE', #1614, 6.500000000000024869, 0.7853981633974488341 ) ;
#74221=CARTESIAN_POINT ( 'NONE',  ( 197.1513938986460062, -147.7221692137691775, 1.978481845683761620 ) ) ;
#74616=CIRCLE ( 'NONE', #83667, 8.500000000000007105 ) ;
#74938=ORIENTED_EDGE ( 'NONE', *, *, #30297, .F. ) ;
#75100=CARTESIAN_POINT ( 'NONE',  ( 200.9306832106270804, -199.2391364535880882, 0.000000000000000000 ) ) ;
#75110=DIRECTION ( 'NONE',  ( -0.000000000000000000, 1.000000000000000000, -0.000000000000000000 ) ) ;
#75199=ORIENTED_EDGE ( 'NONE', *, *, #79173, .F. ) ;
#75250=EDGE_LOOP ( 'NONE', ( #75199, #17858, #61668, #46295, #21282 ) ) ;
#75475=CARTESIAN_POINT ( 'NONE',  ( 208.4306832106270804, -147.7221692137691775, -8.500000000000007105 ) ) ;
#75646=LINE ( 'NONE', #25002, #70017 ) ;
#75854=CARTESIAN_POINT ( 'NONE',  ( 208.4306832106270804, -147.7221692137691775, 8.500000000000007105 ) ) ;
#75878=ORIENTED_EDGE ( 'NONE', *, *, #15862, .T. ) ;
#75951=FACE_OUTER_BOUND ( 'NONE', #23934, .T. ) ;
#75964=AXIS2_PLACEMENT_3D ( 'NONE', #39550, #40032, #17814 ) ;
#76033=CARTESIAN_POINT ( 'NONE',  ( 208.4306832106270804, -198.2391364535880598, 0.000000000000000000 ) ) ;
#76037=DIRECTION ( 'NONE',  ( 0.000000000000000000, 0.000000000000000000, 1.000000000000000000 ) ) ;
#76269=CARTESIAN_POINT ( 'NONE',  ( 201.0776230153480526, -147.7221692137691775, -8.778910157967986905 ) ) ;
#76475=VERTEX_POINT ( 'NONE', #77689 ) ;
#76670=DIRECTION ( 'NONE',  ( 0.000000000000000000, -1.000000000000000000, 0.000000000000000000 ) ) ;
#76676=EDGE_CURVE ( 'NONE', #37419, #20412, #25730, .T. ) ;
#76910=ORIENTED_EDGE ( 'NONE', *, *, #72465, .F. ) ;
#76986=CARTESIAN_POINT ( 'NONE',  ( 212.3569123273291268, -147.7221692137691775, -10.75739200365177695 ) ) ;
#77042=VERTEX_POINT ( 'NONE', #76986 ) ;
#77139=CARTESIAN_POINT ( 'NONE',  ( 208.4306832106270804, -148.7221692137691491, 0.000000000000000000 ) ) ;
#77178=LINE ( 'NONE', #53993, #47339 ) ;
#77226=ORIENTED_EDGE ( 'NONE', *, *, #6030, .F. ) ;
#77438=DIRECTION ( 'NONE',  ( 0.000000000000000000, 0.000000000000000000, 1.000000000000000000 ) ) ;
#77439=CARTESIAN_POINT ( 'NONE',  ( 219.7099725226080977, -142.7221692137691775, -1.978481845683818907 ) ) ;
#77447=VECTOR ( 'NONE', #39059, 1000.000000000000114 ) ;
#77525=AXIS2_PLACEMENT_3D ( 'NONE', #84522, #48537, #77438 ) ;
#77689=CARTESIAN_POINT ( 'NONE',  ( 208.4306832106270804, -198.2391364535880598, -7.500000000000012434 ) ) ;
#77860=ORIENTED_EDGE ( 'NONE', *, *, #1655, .T. ) ;
#77878=ADVANCED_FACE ( 'NONE', ( #2582 ), #39359, .T. ) ;
#77906=EDGE_CURVE ( 'NONE', #20412, #64509, #4657, .T. ) ;
#77981=DIRECTION ( 'NONE',  ( 0.000000000000000000, 0.000000000000000000, 1.000000000000000000 ) ) ;
#77991=ADVANCED_FACE ( 'NONE', ( #39455 ), #74201, .T. ) ;
#78028=LINE ( 'NONE', #56729, #15702 ) ;
#78640=CARTESIAN_POINT ( 'NONE',  ( 212.3569123273291268, -147.7221692137691775, -10.75739200365177695 ) ) ;
#78678=AXIS2_PLACEMENT_3D ( 'NONE', #72010, #7127, #27980 ) ;
#79169=DIRECTION ( 'NONE',  ( 0.000000000000000000, -1.000000000000000000, 0.000000000000000000 ) ) ;
#79173=EDGE_CURVE ( 'NONE', #83213, #64509, #80134, .T. ) ;
#79527=ORIENTED_EDGE ( 'NONE', *, *, #23558, .F. ) ;
#79592=DIRECTION ( 'NONE',  ( 0.000000000000000000, -1.000000000000000000, 0.000000000000000000 ) ) ;
#79683=ORIENTED_EDGE ( 'NONE', *, *, #1655, .F. ) ;
#79915=DIRECTION ( 'NONE',  ( -0.000000000000000000, 1.000000000000000000, -0.000000000000000000 ) ) ;
#80028=CYLINDRICAL_SURFACE ( 'NONE', #8060, 7.500000000000007105 ) ;
#80114=CARTESIAN_POINT ( 'NONE',  ( 208.4306832106270804, -148.7221692137691491, 0.000000000000000000 ) ) ;
#80134=LINE ( 'NONE', #72574, #57889 ) ;
#80366=ORIENTED_EDGE ( 'NONE', *, *, #7541, .F. ) ;
#80958=CARTESIAN_POINT ( 'NONE',  ( 215.7837434059060229, -142.7221692137691775, 8.778910157967997563 ) ) ;
#81055=ADVANCED_FACE ( 'NONE', ( #49283 ), #80028, .T. ) ;
#81466=EDGE_CURVE ( 'NONE', #85835, #45114, #8515, .T. ) ;
#81785=ADVANCED_FACE ( 'NONE', ( #88518 ), #60594, .T. ) ;
#81956=DIRECTION ( 'NONE',  ( 0.000000000000000000, 0.000000000000000000, 1.000000000000000000 ) ) ;
#81972=ORIENTED_EDGE ( 'NONE', *, *, #50919, .F. ) ;
#82438=ADVANCED_FACE ( 'NONE', ( #5162 ), #34037, .F. ) ;
#82570=CARTESIAN_POINT ( 'NONE',  ( 208.4306832106270804, -147.7221692137691775, 0.000000000000000000 ) ) ;
#82850=DIRECTION ( 'NONE',  ( 0.000000000000000000, 0.000000000000000000, 1.000000000000000000 ) ) ;
#82985=CARTESIAN_POINT ( 'NONE',  ( 208.4306832106270804, -124.2391364535881024, 0.000000000000000000 ) ) ;
#83213=VERTEX_POINT ( 'NONE', #7032 ) ;
#83264=ORIENTED_EDGE ( 'NONE', *, *, #68323, .F. ) ;
#83307=VECTOR ( 'NONE', #48462, 1000.000000000000000 ) ;
#83312=DIRECTION ( 'NONE',  ( -0.000000000000000000, 1.000000000000000000, -0.000000000000000000 ) ) ;
#83365=ADVANCED_FACE ( 'NONE', ( #59554 ), #59588, .T. ) ;
#83541=EDGE_LOOP ( 'NONE', ( #32977, #73541, #74938, #19762 ) ) ;
#83604=EDGE_CURVE ( 'NONE', #41385, #45114, #22606, .T. ) ;
#83667=AXIS2_PLACEMENT_3D ( 'NONE', #33171, #62061, #41175 ) ;
#84023=( GEOMETRIC_REPRESENTATION_CONTEXT ( 3 ) GLOBAL_UNCERTAINTY_ASSIGNED_CONTEXT ( ( #40526 ) ) GLOBAL_UNIT_ASSIGNED_CONTEXT ( ( #42925, #86002, #85074 ) ) REPRESENTATION_CONTEXT ( 'NONE', 'WORKASPACE' ) );
#84108=ORIENTED_EDGE ( 'NONE', *, *, #81466, .F. ) ;
#84522=CARTESIAN_POINT ( 'NONE',  ( 208.4306832106270804, -198.2391364535880598, 0.000000000000000000 ) ) ;
#84776=DIRECTION ( 'NONE',  ( -0.7666168903225496489, 0.000000000000000000, 0.6421047760857910847 ) ) ;
#84816=ORIENTED_EDGE ( 'NONE', *, *, #83604, .T. ) ;
#84942=AXIS2_PLACEMENT_3D ( 'NONE', #86274, #14349, #81956 ) ;
#84957=ORIENTED_EDGE ( 'NONE', *, *, #4770, .T. ) ;
#85074=( NAMED_UNIT ( * ) SI_UNIT ( $, .STERADIAN. ) SOLID_ANGLE_UNIT ( ) );
#85120=DIRECTION ( 'NONE',  ( 0.000000000000000000, -1.000000000000000000, 0.000000000000000000 ) ) ;
#85266=CARTESIAN_POINT ( 'NONE',  ( 208.4306832106270804, -199.2391364535880882, 0.000000000000000000 ) ) ;
#85327=CARTESIAN_POINT ( 'NONE',  ( 208.4306832106270804, -148.7221692137691491, 0.000000000000000000 ) ) ;
#85835=VERTEX_POINT ( 'NONE', #72484 ) ;
#85857=ADVANCED_FACE ( 'NONE', ( #6698, #44040 ), #28464, .F. ) ;
#86002=( NAMED_UNIT ( * ) PLANE_ANGLE_UNIT ( ) SI_UNIT ( $, .RADIAN. ) );
#86274=CARTESIAN_POINT ( 'NONE',  ( 208.4306832106270804, -125.2391364535880882, 0.000000000000000000 ) ) ;
#86556=LINE ( 'NONE', #74221, #44749 ) ;
#86650=CIRCLE ( 'NONE', #57959, 7.500000000000012434 ) ;
#86658=VECTOR ( 'NONE', #16556, 1000.000000000000000 ) ;
#86666=DIRECTION ( 'NONE',  ( 1.124465274301078034E-16, 1.000000000000000000, 0.000000000000000000 ) ) ;
#86820=ORIENTED_EDGE ( 'NONE', *, *, #55554, .T. ) ;
#86851=ADVANCED_FACE ( 'NONE', ( #16115 ), #44966, .F. ) ;
#86869=DIRECTION ( 'NONE',  ( 0.000000000000000000, -0.000000000000000000, -1.000000000000000000 ) ) ;
#86922=DIRECTION ( 'NONE',  ( 8.659560562354958743E-17, 0.7071067811865453523, -0.7071067811865496822 ) ) ;
#86979=PLANE ( 'NONE',  #44114 ) ;
#87134=LINE ( 'NONE', #93315, #60230 ) ;
#87872=FACE_OUTER_BOUND ( 'NONE', #83541, .T. ) ;
#87964=VECTOR ( 'NONE', #21161, 1000.000000000000114 ) ;
#87966=CIRCLE ( 'NONE', #7824, 7.500000000000012434 ) ;
#88072=ORIENTED_EDGE ( 'NONE', *, *, #72465, .T. ) ;
#88080=DIRECTION ( 'NONE',  ( 0.000000000000000000, 0.000000000000000000, -1.000000000000000000 ) ) ;
#88143=VERTEX_POINT ( 'NONE', #40649 ) ;
#88194=VERTEX_POINT ( 'NONE', #25083 ) ;
#88518=FACE_OUTER_BOUND ( 'NONE', #25441, .T. ) ;
#88559=CARTESIAN_POINT ( 'NONE',  ( 208.4306832106270804, -148.7221692137691491, -7.500000000000012434 ) ) ;
#88679=ORIENTED_EDGE ( 'NONE', *, *, #45323, .F. ) ;
#88730=DIRECTION ( 'NONE',  ( 0.000000000000000000, 0.000000000000000000, 1.000000000000000000 ) ) ;
#89032=DIRECTION ( 'NONE',  ( 1.124465274301078034E-16, 1.000000000000000000, 0.000000000000000000 ) ) ;
#89716=VECTOR ( 'NONE', #67661, 1000.000000000000000 ) ;
#90091=DIRECTION ( 'NONE',  ( 0.000000000000000000, -1.000000000000000000, 0.000000000000000000 ) ) ;
#90125=ORIENTED_EDGE ( 'NONE', *, *, #76676, .F. ) ;
#90135=MANIFOLD_SOLID_BREP ( 'Chamfer2', #5316 ) ;
#90166=VERTEX_POINT ( 'NONE', #64744 ) ;
#90459=ORIENTED_EDGE ( 'NONE', *, *, #22911, .F. ) ;
#90592=DIRECTION ( 'NONE',  ( 1.124465274301078034E-16, 1.000000000000000000, 0.000000000000000000 ) ) ;
#90686=DIRECTION ( 'NONE',  ( 0.7666168903225505371, 0.000000000000000000, -0.6421047760857900855 ) ) ;
#90762=ORIENTED_EDGE ( 'NONE', *, *, #50406, .T. ) ;
#90811=ORIENTED_EDGE ( 'NONE', *, *, #67295, .F. ) ;
#90959=CARTESIAN_POINT ( 'NONE',  ( 0.000000000000000000, 0.000000000000000000, 0.000000000000000000 ) ) ;
#90984=CARTESIAN_POINT ( 'NONE',  ( 212.3569123273291268, -147.7221692137691775, -10.75739200365177695 ) ) ;
#91014=DIRECTION ( 'NONE',  ( 0.9849620900324523864, 0.000000000000000000, -0.1727706028203384037 ) ) ;
#91140=DIRECTION ( 'NONE',  ( -0.000000000000000000, 1.000000000000000000, -0.000000000000000000 ) ) ;
#91473=EDGE_LOOP ( 'NONE', ( #14171, #79527, #81972, #66135, #46238, #84108 ) ) ;
#91610=DIRECTION ( 'NONE',  ( 1.124465274301078034E-16, 1.000000000000000000, 0.000000000000000000 ) ) ;
#91976=EDGE_CURVE ( 'NONE', #71100, #88143, #86556, .T. ) ;
#92104=CIRCLE ( 'NONE', #48300, 6.499999999999977796 ) ;
#92114=DIRECTION ( 'NONE',  ( -1.124465274301078034E-16, -1.000000000000000000, -0.000000000000000000 ) ) ;
#92381=ORIENTED_EDGE ( 'NONE', *, *, #9285, .F. ) ;
#92401=EDGE_LOOP ( 'NONE', ( #90762, #36420 ) ) ;
#92685=CARTESIAN_POINT ( 'NONE',  ( 197.1513938986460062, -147.7221692137691775, 1.978481845683761620 ) ) ;
#93315=CARTESIAN_POINT ( 'NONE',  ( 200.9306832106270804, -199.2391364535880882, 0.000000000000000000 ) ) ;
#93472=ORIENTED_EDGE ( 'NONE', *, *, #67295, .T. ) ;
#93585=VERTEX_POINT ( 'NONE', #75854 ) ;
#93746=COLOUR_RGB('Grey',0.48,0.52,0.57);
#93747=FILL_AREA_STYLE_COLOUR('',#93746);
#93748=FILL_AREA_STYLE('',(#93747));
#93749=SURFACE_STYLE_FILL_AREA(#93748);
#93750=SURFACE_SIDE_STYLE('',(#93749));
#93751=SURFACE_STYLE_USAGE(.BOTH.,#93750);
#93752=PRESENTATION_STYLE_ASSIGNMENT((#93751));
ENDSEC;
END-ISO-10303-21;
